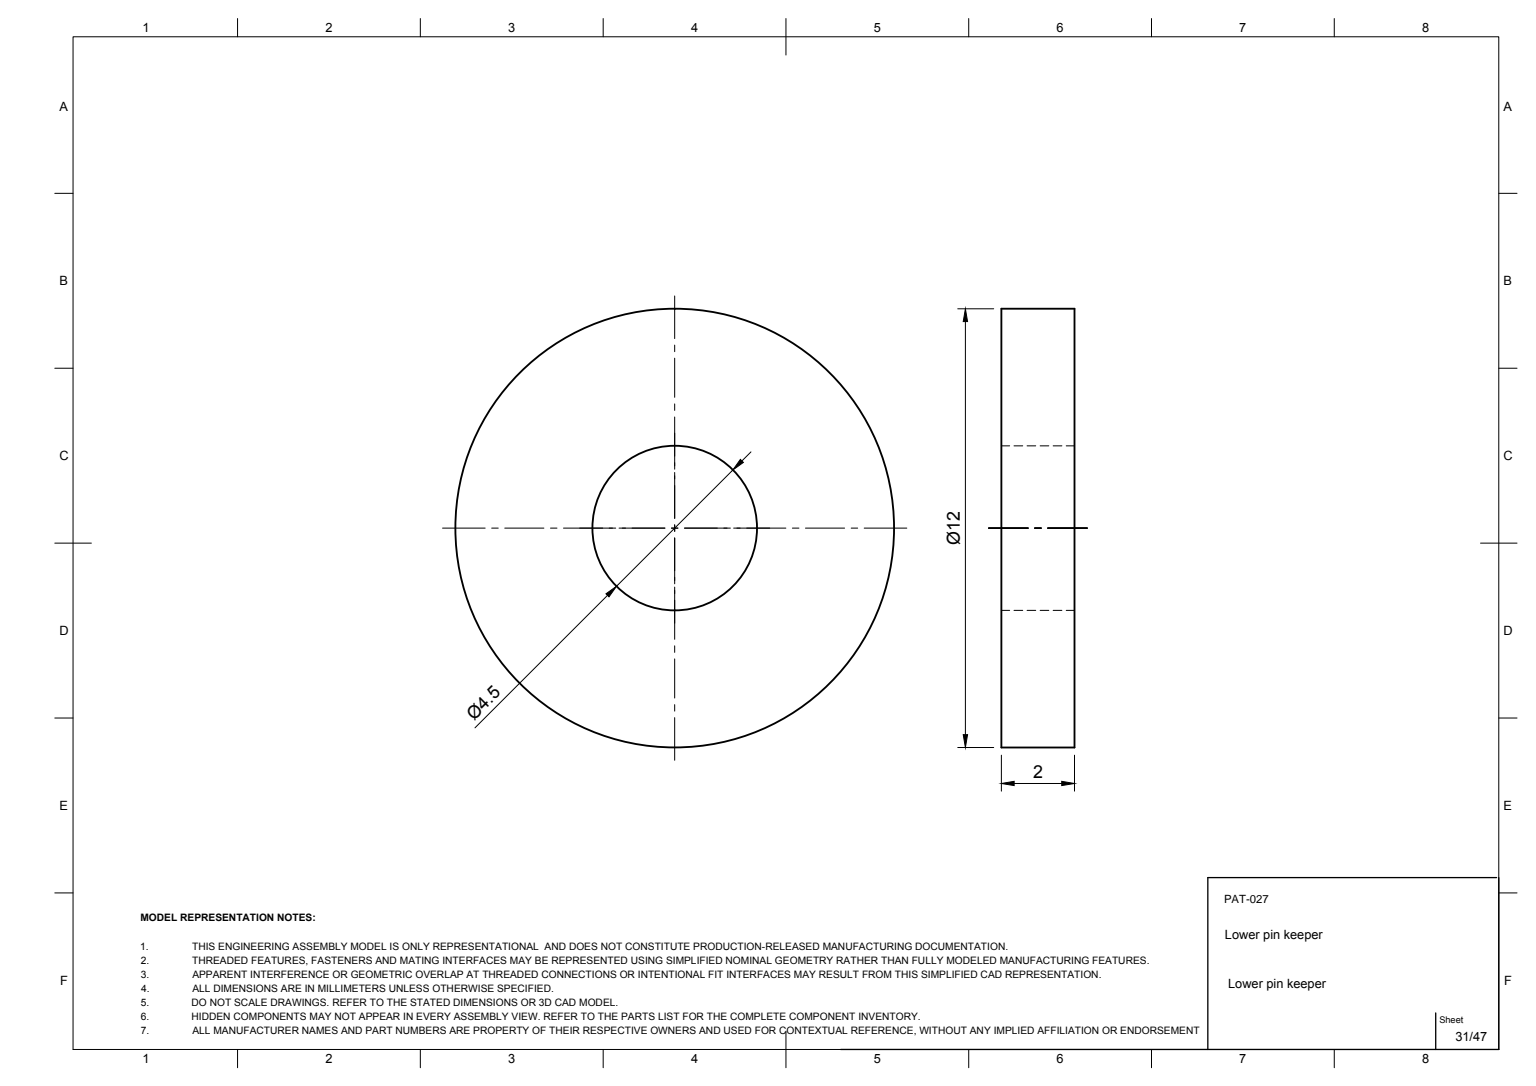
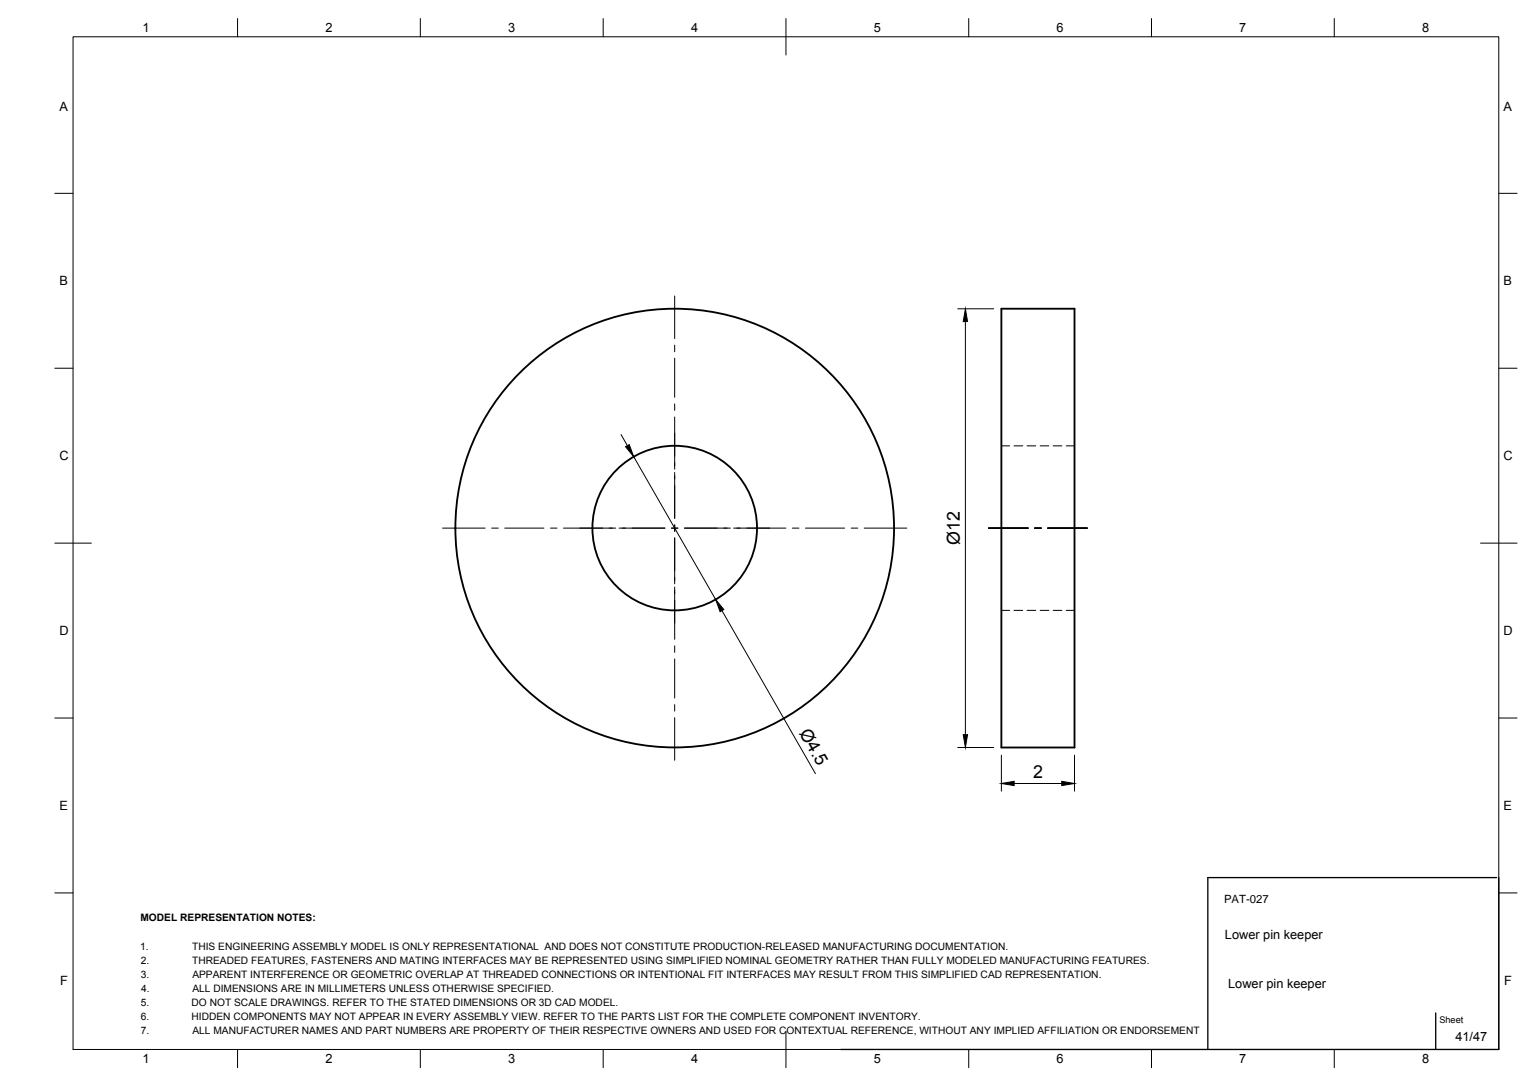
ISO-10303-21;
HEADER;
/* Generated by software containing ST-Developer
 * from STEP Tools, Inc. (www.steptools.com) 
 */

FILE_DESCRIPTION(
/* description */ ('Crank-driven oscillating fan base (mechanism only)'),

/* implementation_level */ '2;1');

FILE_NAME(
/* name */ 'Lower pin keeper.step',
/* time_stamp */ '2026-10-28T03:25:00-07:00',
/* author */ (''),
/* organization */ (''),
/* preprocessor_version */ 'ST-DEVELOPER v20.2',
/* originating_system */ 'Autodesk Translation Framework v15.17.0.0',
/* authorisation */ '');

FILE_SCHEMA (('AUTOMOTIVE_DESIGN { 1 0 10303 214 3 1 1 }'));
ENDSEC;

DATA;
#10=MECHANICAL_DESIGN_GEOMETRIC_PRESENTATION_REPRESENTATION('',(#468),#11916);
#380=SHAPE_REPRESENTATION_RELATIONSHIP('SRR','None',#12106,#420);
#420=ADVANCED_BREP_SHAPE_REPRESENTATION('',(#515),#11897);
#468=STYLED_ITEM('',(#12375),#515);
#515=MANIFOLD_SOLID_BREP('Body1',#6099);
#644=FACE_BOUND('',#1613,.T.);
#645=FACE_BOUND('',#1615,.T.);
#802=PLANE('',#7096);
#803=PLANE('',#7097);
#1121=FACE_OUTER_BOUND('',#1610,.T.);
#1122=FACE_OUTER_BOUND('',#1611,.T.);
#1123=FACE_OUTER_BOUND('',#1612,.T.);
#1124=FACE_OUTER_BOUND('',#1614,.T.);
#1610=EDGE_LOOP('',(#5024,#5025,#5026,#5027));
#1611=EDGE_LOOP('',(#5028,#5029,#5030,#5031));
#1612=EDGE_LOOP('',(#5032));
#1613=EDGE_LOOP('',(#5033));
#1614=EDGE_LOOP('',(#5034));
#1615=EDGE_LOOP('',(#5035));
#1977=LINE('',#11115,#2310);
#1978=LINE('',#11121,#2311);
#2310=VECTOR('',#8656,0.225);
#2311=VECTOR('',#8663,0.6);
#2727=CIRCLE('',#7091,0.225);
#2728=CIRCLE('',#7092,0.225);
#2729=CIRCLE('',#7094,0.6);
#2730=CIRCLE('',#7095,0.6);
#3158=VERTEX_POINT('',#11112);
#3159=VERTEX_POINT('',#11114);
#3160=VERTEX_POINT('',#11118);
#3161=VERTEX_POINT('',#11120);
#3807=EDGE_CURVE('',#3158,#3158,#2727,.T.);
#3808=EDGE_CURVE('',#3158,#3159,#1977,.T.);
#3809=EDGE_CURVE('',#3159,#3159,#2728,.T.);
#3810=EDGE_CURVE('',#3160,#3160,#2729,.T.);
#3811=EDGE_CURVE('',#3160,#3161,#1978,.T.);
#3812=EDGE_CURVE('',#3161,#3161,#2730,.T.);
#5024=ORIENTED_EDGE('',*,*,#3807,.F.);
#5025=ORIENTED_EDGE('',*,*,#3808,.T.);
#5026=ORIENTED_EDGE('',*,*,#3809,.T.);
#5027=ORIENTED_EDGE('',*,*,#3808,.F.);
#5028=ORIENTED_EDGE('',*,*,#3810,.F.);
#5029=ORIENTED_EDGE('',*,*,#3811,.T.);
#5030=ORIENTED_EDGE('',*,*,#3812,.T.);
#5031=ORIENTED_EDGE('',*,*,#3811,.F.);
#5032=ORIENTED_EDGE('',*,*,#3810,.T.);
#5033=ORIENTED_EDGE('',*,*,#3807,.T.);
#5034=ORIENTED_EDGE('',*,*,#3812,.F.);
#5035=ORIENTED_EDGE('',*,*,#3809,.F.);
#5646=CYLINDRICAL_SURFACE('',#7090,0.225);
#5647=CYLINDRICAL_SURFACE('',#7093,0.6);
#5927=ADVANCED_FACE('',(#1121),#5646,.F.);
#5928=ADVANCED_FACE('',(#1122),#5647,.T.);
#5929=ADVANCED_FACE('',(#1123,#644),#802,.T.);
#5930=ADVANCED_FACE('',(#1124,#645),#803,.F.);
#6099=CLOSED_SHELL('',(#5927,#5928,#5929,#5930));
#7089=AXIS2_PLACEMENT_3D('',#11110,#8650,#8651);
#7090=AXIS2_PLACEMENT_3D('',#11111,#8652,#8653);
#7091=AXIS2_PLACEMENT_3D('',#11113,#8654,#8655);
#7092=AXIS2_PLACEMENT_3D('',#11116,#8657,#8658);
#7093=AXIS2_PLACEMENT_3D('',#11117,#8659,#8660);
#7094=AXIS2_PLACEMENT_3D('',#11119,#8661,#8662);
#7095=AXIS2_PLACEMENT_3D('',#11122,#8664,#8665);
#7096=AXIS2_PLACEMENT_3D('',#11123,#8666,#8667);
#7097=AXIS2_PLACEMENT_3D('',#11124,#8668,#8669);
#8650=DIRECTION('axis',(0.,0.,1.));
#8651=DIRECTION('refdir',(1.,0.,0.));
#8652=DIRECTION('center_axis',(0.,0.,1.));
#8653=DIRECTION('ref_axis',(1.,0.,0.));
#8654=DIRECTION('center_axis',(0.,0.,-1.));
#8655=DIRECTION('ref_axis',(1.,0.,0.));
#8656=DIRECTION('',(0.,0.,-1.));
#8657=DIRECTION('center_axis',(0.,0.,-1.));
#8658=DIRECTION('ref_axis',(1.,0.,0.));
#8659=DIRECTION('center_axis',(0.,0.,1.));
#8660=DIRECTION('ref_axis',(1.,0.,0.));
#8661=DIRECTION('center_axis',(0.,0.,1.));
#8662=DIRECTION('ref_axis',(1.,0.,0.));
#8663=DIRECTION('',(0.,0.,-1.));
#8664=DIRECTION('center_axis',(0.,0.,1.));
#8665=DIRECTION('ref_axis',(1.,0.,0.));
#8666=DIRECTION('center_axis',(0.,0.,1.));
#8667=DIRECTION('ref_axis',(1.,0.,0.));
#8668=DIRECTION('center_axis',(0.,0.,1.));
#8669=DIRECTION('ref_axis',(1.,0.,0.));
#11110=CARTESIAN_POINT('',(0.,0.,0.));
#11111=CARTESIAN_POINT('Origin',(-0.429855350392604,2.61349944954989,6.));
#11112=CARTESIAN_POINT('',(-0.654855350392604,2.61349944954989,6.2));
#11113=CARTESIAN_POINT('Origin',(-0.429855350392604,2.61349944954989,6.2));
#11114=CARTESIAN_POINT('',(-0.654855350392604,2.61349944954989,6.));
#11115=CARTESIAN_POINT('',(-0.654855350392604,2.61349944954989,6.));
#11116=CARTESIAN_POINT('Origin',(-0.429855350392604,2.61349944954989,6.));
#11117=CARTESIAN_POINT('Origin',(-0.429855350392604,2.61349944954989,6.));
#11118=CARTESIAN_POINT('',(-1.0298553503926,2.61349944954989,6.2));
#11119=CARTESIAN_POINT('Origin',(-0.429855350392604,2.61349944954989,6.2));
#11120=CARTESIAN_POINT('',(-1.0298553503926,2.61349944954989,6.));
#11121=CARTESIAN_POINT('',(-1.0298553503926,2.61349944954989,6.));
#11122=CARTESIAN_POINT('Origin',(-0.429855350392604,2.61349944954989,6.));
#11123=CARTESIAN_POINT('Origin',(-0.429855350392604,2.61349944954989,6.2));
#11124=CARTESIAN_POINT('Origin',(-0.429855350392604,2.61349944954989,6.));
#11850=UNCERTAINTY_MEASURE_WITH_UNIT(LENGTH_MEASURE(0.001),#11917,
'DISTANCE_ACCURACY_VALUE',
'Maximum model space distance between geometric entities at asserted c
onnectivities');
#11869=UNCERTAINTY_MEASURE_WITH_UNIT(LENGTH_MEASURE(0.001),#11917,
'DISTANCE_ACCURACY_VALUE',
'Maximum model space distance between geometric entities at asserted c
onnectivities');
#11897=(
GEOMETRIC_REPRESENTATION_CONTEXT(3)
GLOBAL_UNCERTAINTY_ASSIGNED_CONTEXT((#11850))
GLOBAL_UNIT_ASSIGNED_CONTEXT((#11917,#11919,#11920))
REPRESENTATION_CONTEXT('','3D')
);
#11916=(
GEOMETRIC_REPRESENTATION_CONTEXT(3)
GLOBAL_UNCERTAINTY_ASSIGNED_CONTEXT((#11869))
GLOBAL_UNIT_ASSIGNED_CONTEXT((#11917,#11919,#11920))
REPRESENTATION_CONTEXT('','3D')
);
#11917=(
LENGTH_UNIT()
NAMED_UNIT(*)
SI_UNIT(.CENTI.,.METRE.)
);
#11919=(
NAMED_UNIT(*)
PLANE_ANGLE_UNIT()
SI_UNIT($,.RADIAN.)
);
#11920=(
NAMED_UNIT(*)
SI_UNIT($,.STERADIAN.)
SOLID_ANGLE_UNIT()
);
#11948=SHAPE_DEFINITION_REPRESENTATION(#11999,#12106);
#11999=PRODUCT_DEFINITION_SHAPE('',$,#12153);
#12106=SHAPE_REPRESENTATION('',(#7089),#11897);
#12125=PRODUCT_DEFINITION_CONTEXT('part definition',#12265,'design');
#12153=PRODUCT_DEFINITION('Lower pin keeper','Lower pin keeper',#12199,
#12125);
#12199=PRODUCT_DEFINITION_FORMATION('',$,#12294);
#12265=APPLICATION_CONTEXT(
'Core Data for Automotive Mechanical Design Process');
#12266=PRODUCT_CONTEXT('part definition',#12265,'mechanical');
#12294=PRODUCT('Lower pin keeper','Lower pin keeper','Lower pin keeper',
(#12266));
#12369=COLOUR_RGB('Grey',0.48,0.52,0.57);
#12370=FILL_AREA_STYLE_COLOUR('',#12369);
#12371=FILL_AREA_STYLE('',(#12370));
#12372=SURFACE_STYLE_FILL_AREA(#12371);
#12373=SURFACE_SIDE_STYLE('',(#12372));
#12374=SURFACE_STYLE_USAGE(.BOTH.,#12373);
#12375=PRESENTATION_STYLE_ASSIGNMENT((#12374));
ENDSEC;
END-ISO-10303-21;
